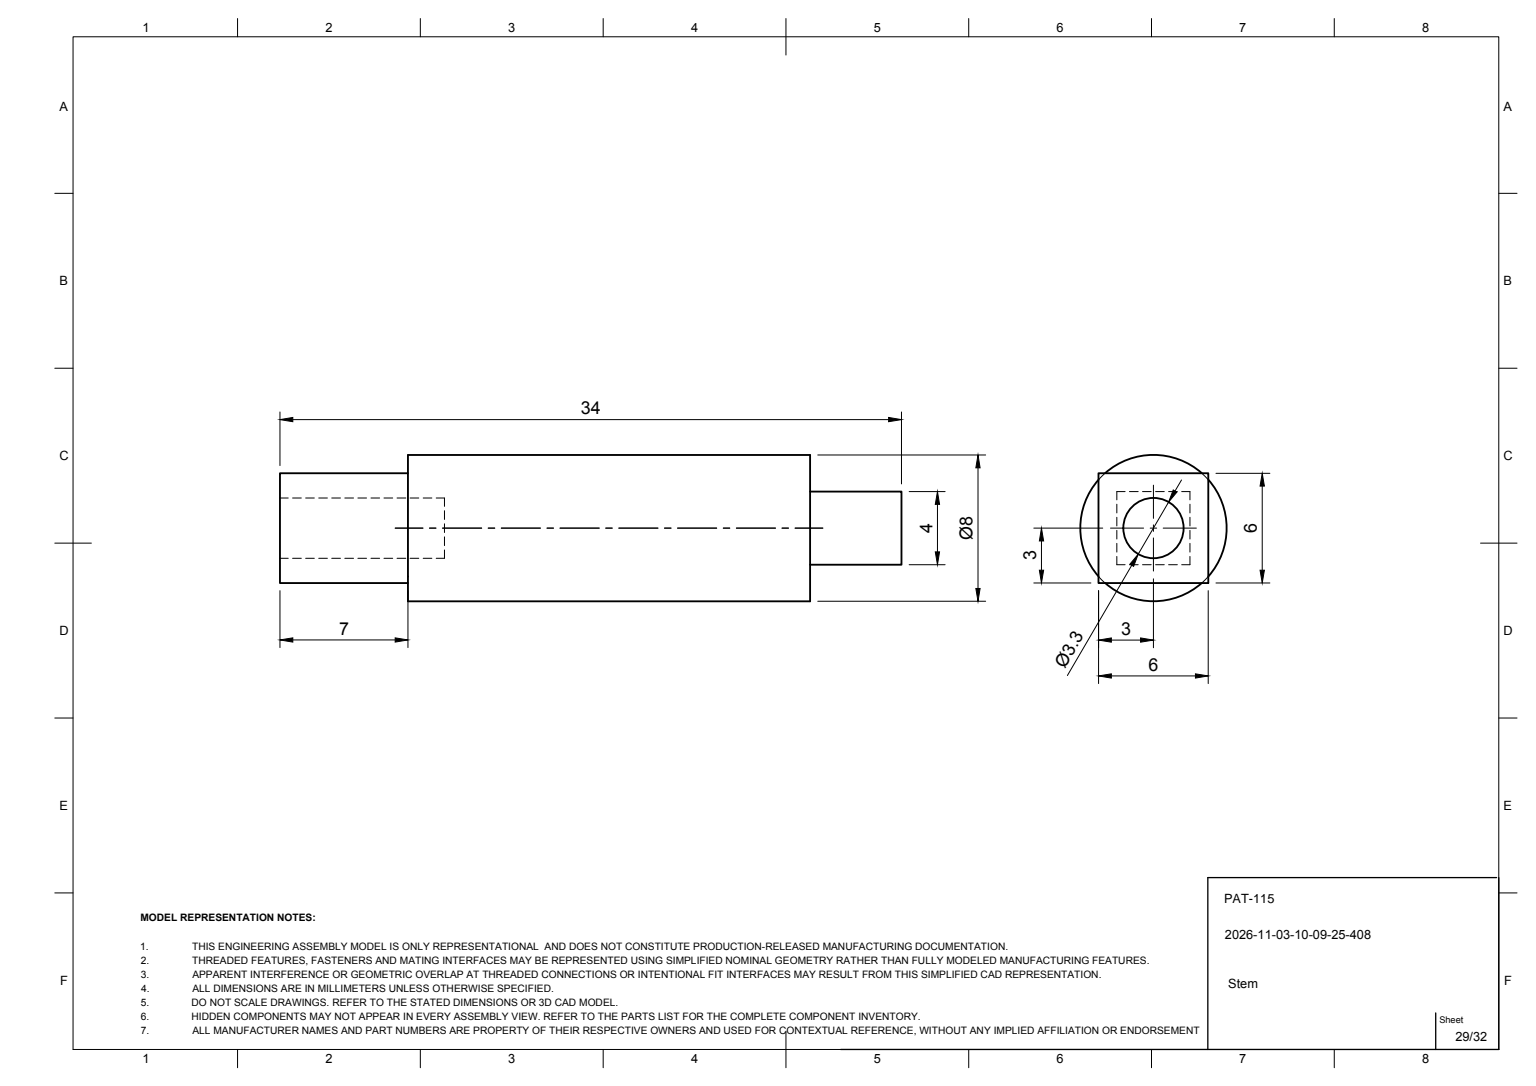
ISO-10303-21;
HEADER;
/* Generated by software containing ST-Developer
 * from STEP Tools, Inc. (www.steptools.com) 
 */

FILE_DESCRIPTION(
/* description */ ('Union bypass pipe loop'),
/* implementation_level */ '2;1');

FILE_NAME(
/* name */ 'Stem.step',
/* time_stamp */ '2026-10-27T21:00:29-07:00',
/* author */ (''),
/* organization */ (''),
/* preprocessor_version */ 'ST-DEVELOPER v20.2',
/* originating_system */ 'Autodesk Translation Framework v15.17.0.0',
/* authorisation */ '');

FILE_SCHEMA (('AUTOMOTIVE_DESIGN { 1 0 10303 214 3 1 1 }'));
ENDSEC;

DATA;
#10=MECHANICAL_DESIGN_GEOMETRIC_PRESENTATION_REPRESENTATION('',(#472),#10095);
#408=SHAPE_REPRESENTATION_RELATIONSHIP('SRR','None',#10278,#440);
#440=ADVANCED_BREP_SHAPE_REPRESENTATION('',(#501),#10090);
#472=STYLED_ITEM('',(#10493),#501);
#501=MANIFOLD_SOLID_BREP('Body1',#5546);
#628=FACE_BOUND('',#1569,.T.);
#629=FACE_BOUND('',#1581,.T.);
#786=PLANE('',#6529);
#787=PLANE('',#6530);
#788=PLANE('',#6532);
#789=PLANE('',#6534);
#790=PLANE('',#6536);
#791=PLANE('',#6538);
#792=PLANE('',#6539);
#793=PLANE('',#6540);
#794=PLANE('',#6541);
#795=PLANE('',#6542);
#796=PLANE('',#6543);
#797=PLANE('',#6545);
#798=PLANE('',#6548);
#799=PLANE('',#6550);
#800=PLANE('',#6552);
#801=PLANE('',#6553);
#802=PLANE('',#6554);
#803=PLANE('',#6555);
#804=PLANE('',#6556);
#805=PLANE('',#6559);
#1109=FACE_OUTER_BOUND('',#1558,.T.);
#1110=FACE_OUTER_BOUND('',#1559,.T.);
#1111=FACE_OUTER_BOUND('',#1560,.T.);
#1112=FACE_OUTER_BOUND('',#1561,.T.);
#1113=FACE_OUTER_BOUND('',#1562,.T.);
#1114=FACE_OUTER_BOUND('',#1563,.T.);
#1115=FACE_OUTER_BOUND('',#1564,.T.);
#1116=FACE_OUTER_BOUND('',#1565,.T.);
#1117=FACE_OUTER_BOUND('',#1566,.T.);
#1118=FACE_OUTER_BOUND('',#1567,.T.);
#1119=FACE_OUTER_BOUND('',#1568,.T.);
#1120=FACE_OUTER_BOUND('',#1570,.T.);
#1121=FACE_OUTER_BOUND('',#1571,.T.);
#1122=FACE_OUTER_BOUND('',#1572,.T.);
#1123=FACE_OUTER_BOUND('',#1573,.T.);
#1124=FACE_OUTER_BOUND('',#1574,.T.);
#1125=FACE_OUTER_BOUND('',#1575,.T.);
#1126=FACE_OUTER_BOUND('',#1576,.T.);
#1127=FACE_OUTER_BOUND('',#1577,.T.);
#1128=FACE_OUTER_BOUND('',#1578,.T.);
#1129=FACE_OUTER_BOUND('',#1579,.T.);
#1130=FACE_OUTER_BOUND('',#1580,.T.);
#1558=EDGE_LOOP('',(#4844,#4845,#4846,#4847));
#1559=EDGE_LOOP('',(#4848));
#1560=EDGE_LOOP('',(#4849,#4850,#4851));
#1561=EDGE_LOOP('',(#4852,#4853,#4854));
#1562=EDGE_LOOP('',(#4855,#4856,#4857));
#1563=EDGE_LOOP('',(#4858,#4859,#4860));
#1564=EDGE_LOOP('',(#4861,#4862,#4863,#4864,#4865,#4866));
#1565=EDGE_LOOP('',(#4867,#4868,#4869,#4870,#4871,#4872));
#1566=EDGE_LOOP('',(#4873,#4874,#4875,#4876,#4877,#4878));
#1567=EDGE_LOOP('',(#4879,#4880,#4881,#4882,#4883,#4884));
#1568=EDGE_LOOP('',(#4885,#4886,#4887,#4888));
#1569=EDGE_LOOP('',(#4889));
#1570=EDGE_LOOP('',(#4890,#4891));
#1571=EDGE_LOOP('',(#4892,#4893,#4894));
#1572=EDGE_LOOP('',(#4895,#4896));
#1573=EDGE_LOOP('',(#4897,#4898));
#1574=EDGE_LOOP('',(#4899,#4900,#4901,#4902));
#1575=EDGE_LOOP('',(#4903,#4904,#4905,#4906));
#1576=EDGE_LOOP('',(#4907,#4908,#4909,#4910));
#1577=EDGE_LOOP('',(#4911,#4912,#4913,#4914));
#1578=EDGE_LOOP('',(#4915,#4916,#4917,#4918));
#1579=EDGE_LOOP('',(#4919,#4920,#4921,#4922,#4923,#4924,#4925,#4926,#4927,
#4928,#4929,#4930));
#1580=EDGE_LOOP('',(#4931));
#1581=EDGE_LOOP('',(#4932,#4933,#4934,#4935));
#1904=LINE('',#9763,#2280);
#1905=LINE('',#9771,#2281);
#1906=LINE('',#9772,#2282);
#1907=LINE('',#9778,#2283);
#1908=LINE('',#9779,#2284);
#1909=LINE('',#9785,#2285);
#1910=LINE('',#9786,#2286);
#1911=LINE('',#9792,#2287);
#1912=LINE('',#9793,#2288);
#1913=LINE('',#9795,#2289);
#1914=LINE('',#9797,#2290);
#1915=LINE('',#9799,#2291);
#1916=LINE('',#9800,#2292);
#1917=LINE('',#9802,#2293);
#1918=LINE('',#9804,#2294);
#1919=LINE('',#9805,#2295);
#1920=LINE('',#9807,#2296);
#1921=LINE('',#9809,#2297);
#1922=LINE('',#9810,#2298);
#1923=LINE('',#9812,#2299);
#1924=LINE('',#9813,#2300);
#1925=LINE('',#9828,#2301);
#1926=LINE('',#9830,#2302);
#1927=LINE('',#9832,#2303);
#1928=LINE('',#9833,#2304);
#1929=LINE('',#9836,#2305);
#1930=LINE('',#9838,#2306);
#1931=LINE('',#9839,#2307);
#1932=LINE('',#9842,#2308);
#1933=LINE('',#9844,#2309);
#1934=LINE('',#9845,#2310);
#1935=LINE('',#9847,#2311);
#1936=LINE('',#9848,#2312);
#1937=LINE('',#9852,#2313);
#2280=VECTOR('',#8146,0.165);
#2281=VECTOR('',#8155,1.);
#2282=VECTOR('',#8156,1.);
#2283=VECTOR('',#8161,1.);
#2284=VECTOR('',#8162,1.);
#2285=VECTOR('',#8167,1.);
#2286=VECTOR('',#8168,1.);
#2287=VECTOR('',#8173,1.);
#2288=VECTOR('',#8174,1.);
#2289=VECTOR('',#8177,1.);
#2290=VECTOR('',#8178,1.);
#2291=VECTOR('',#8179,1.);
#2292=VECTOR('',#8180,1.);
#2293=VECTOR('',#8183,1.);
#2294=VECTOR('',#8184,1.);
#2295=VECTOR('',#8185,1.);
#2296=VECTOR('',#8188,1.);
#2297=VECTOR('',#8189,1.);
#2298=VECTOR('',#8190,1.);
#2299=VECTOR('',#8193,1.);
#2300=VECTOR('',#8194,1.);
#2301=VECTOR('',#8217,1.);
#2302=VECTOR('',#8218,1.);
#2303=VECTOR('',#8219,1.);
#2304=VECTOR('',#8220,1.);
#2305=VECTOR('',#8223,1.);
#2306=VECTOR('',#8224,1.);
#2307=VECTOR('',#8225,1.);
#2308=VECTOR('',#8228,1.);
#2309=VECTOR('',#8229,1.);
#2310=VECTOR('',#8230,1.);
#2311=VECTOR('',#8233,1.);
#2312=VECTOR('',#8234,1.);
#2313=VECTOR('',#8239,0.4);
#2607=CIRCLE('',#6527,0.165);
#2608=CIRCLE('',#6528,0.165);
#2609=CIRCLE('',#6531,0.4);
#2610=CIRCLE('',#6533,0.4);
#2611=CIRCLE('',#6535,0.4);
#2612=CIRCLE('',#6537,0.4);
#2613=CIRCLE('',#6544,0.4);
#2614=CIRCLE('',#6546,0.4);
#2615=CIRCLE('',#6547,0.4);
#2616=CIRCLE('',#6549,0.4);
#2617=CIRCLE('',#6551,0.4);
#2618=CIRCLE('',#6558,0.4);
#2992=VERTEX_POINT('',#9760);
#2993=VERTEX_POINT('',#9762);
#2994=VERTEX_POINT('',#9767);
#2995=VERTEX_POINT('',#9768);
#2996=VERTEX_POINT('',#9770);
#2997=VERTEX_POINT('',#9774);
#2998=VERTEX_POINT('',#9775);
#2999=VERTEX_POINT('',#9777);
#3000=VERTEX_POINT('',#9781);
#3001=VERTEX_POINT('',#9782);
#3002=VERTEX_POINT('',#9784);
#3003=VERTEX_POINT('',#9788);
#3004=VERTEX_POINT('',#9789);
#3005=VERTEX_POINT('',#9791);
#3006=VERTEX_POINT('',#9796);
#3007=VERTEX_POINT('',#9798);
#3008=VERTEX_POINT('',#9803);
#3009=VERTEX_POINT('',#9808);
#3010=VERTEX_POINT('',#9818);
#3011=VERTEX_POINT('',#9826);
#3012=VERTEX_POINT('',#9827);
#3013=VERTEX_POINT('',#9829);
#3014=VERTEX_POINT('',#9831);
#3015=VERTEX_POINT('',#9835);
#3016=VERTEX_POINT('',#9837);
#3017=VERTEX_POINT('',#9841);
#3018=VERTEX_POINT('',#9843);
#3019=VERTEX_POINT('',#9851);
#3620=EDGE_CURVE('',#2992,#2992,#2607,.T.);
#3621=EDGE_CURVE('',#2992,#2993,#1904,.T.);
#3622=EDGE_CURVE('',#2993,#2993,#2608,.T.);
#3623=EDGE_CURVE('',#2994,#2995,#2609,.T.);
#3624=EDGE_CURVE('',#2996,#2995,#1905,.T.);
#3625=EDGE_CURVE('',#2994,#2996,#1906,.T.);
#3626=EDGE_CURVE('',#2997,#2998,#2610,.T.);
#3627=EDGE_CURVE('',#2999,#2998,#1907,.T.);
#3628=EDGE_CURVE('',#2997,#2999,#1908,.T.);
#3629=EDGE_CURVE('',#3000,#3001,#2611,.T.);
#3630=EDGE_CURVE('',#3002,#3001,#1909,.T.);
#3631=EDGE_CURVE('',#3000,#3002,#1910,.T.);
#3632=EDGE_CURVE('',#3003,#3004,#2612,.T.);
#3633=EDGE_CURVE('',#3005,#3004,#1911,.T.);
#3634=EDGE_CURVE('',#3003,#3005,#1912,.T.);
#3635=EDGE_CURVE('',#2994,#3004,#1913,.T.);
#3636=EDGE_CURVE('',#2996,#3006,#1914,.T.);
#3637=EDGE_CURVE('',#3007,#3006,#1915,.T.);
#3638=EDGE_CURVE('',#3005,#3007,#1916,.T.);
#3639=EDGE_CURVE('',#3003,#3001,#1917,.T.);
#3640=EDGE_CURVE('',#3008,#3007,#1918,.T.);
#3641=EDGE_CURVE('',#3002,#3008,#1919,.T.);
#3642=EDGE_CURVE('',#3000,#2998,#1920,.T.);
#3643=EDGE_CURVE('',#3009,#3008,#1921,.T.);
#3644=EDGE_CURVE('',#2999,#3009,#1922,.T.);
#3645=EDGE_CURVE('',#2997,#2995,#1923,.T.);
#3646=EDGE_CURVE('',#3006,#3009,#1924,.T.);
#3647=EDGE_CURVE('',#2998,#3000,#2613,.T.);
#3648=EDGE_CURVE('',#2995,#3010,#2614,.T.);
#3649=EDGE_CURVE('',#3010,#2997,#2615,.T.);
#3650=EDGE_CURVE('',#3004,#2994,#2616,.T.);
#3651=EDGE_CURVE('',#3001,#3003,#2617,.T.);
#3652=EDGE_CURVE('',#3011,#3012,#1925,.T.);
#3653=EDGE_CURVE('',#3012,#3013,#1926,.T.);
#3654=EDGE_CURVE('',#3014,#3013,#1927,.T.);
#3655=EDGE_CURVE('',#3011,#3014,#1928,.T.);
#3656=EDGE_CURVE('',#3015,#3011,#1929,.T.);
#3657=EDGE_CURVE('',#3016,#3014,#1930,.T.);
#3658=EDGE_CURVE('',#3015,#3016,#1931,.T.);
#3659=EDGE_CURVE('',#3017,#3015,#1932,.T.);
#3660=EDGE_CURVE('',#3018,#3016,#1933,.T.);
#3661=EDGE_CURVE('',#3017,#3018,#1934,.T.);
#3662=EDGE_CURVE('',#3012,#3017,#1935,.T.);
#3663=EDGE_CURVE('',#3013,#3018,#1936,.T.);
#3664=EDGE_CURVE('',#3010,#3019,#1937,.T.);
#3665=EDGE_CURVE('',#3019,#3019,#2618,.T.);
#4844=ORIENTED_EDGE('',*,*,#3620,.F.);
#4845=ORIENTED_EDGE('',*,*,#3621,.T.);
#4846=ORIENTED_EDGE('',*,*,#3622,.F.);
#4847=ORIENTED_EDGE('',*,*,#3621,.F.);
#4848=ORIENTED_EDGE('',*,*,#3620,.T.);
#4849=ORIENTED_EDGE('',*,*,#3623,.T.);
#4850=ORIENTED_EDGE('',*,*,#3624,.F.);
#4851=ORIENTED_EDGE('',*,*,#3625,.F.);
#4852=ORIENTED_EDGE('',*,*,#3626,.T.);
#4853=ORIENTED_EDGE('',*,*,#3627,.F.);
#4854=ORIENTED_EDGE('',*,*,#3628,.F.);
#4855=ORIENTED_EDGE('',*,*,#3629,.T.);
#4856=ORIENTED_EDGE('',*,*,#3630,.F.);
#4857=ORIENTED_EDGE('',*,*,#3631,.F.);
#4858=ORIENTED_EDGE('',*,*,#3632,.T.);
#4859=ORIENTED_EDGE('',*,*,#3633,.F.);
#4860=ORIENTED_EDGE('',*,*,#3634,.F.);
#4861=ORIENTED_EDGE('',*,*,#3633,.T.);
#4862=ORIENTED_EDGE('',*,*,#3635,.F.);
#4863=ORIENTED_EDGE('',*,*,#3625,.T.);
#4864=ORIENTED_EDGE('',*,*,#3636,.T.);
#4865=ORIENTED_EDGE('',*,*,#3637,.F.);
#4866=ORIENTED_EDGE('',*,*,#3638,.F.);
#4867=ORIENTED_EDGE('',*,*,#3630,.T.);
#4868=ORIENTED_EDGE('',*,*,#3639,.F.);
#4869=ORIENTED_EDGE('',*,*,#3634,.T.);
#4870=ORIENTED_EDGE('',*,*,#3638,.T.);
#4871=ORIENTED_EDGE('',*,*,#3640,.F.);
#4872=ORIENTED_EDGE('',*,*,#3641,.F.);
#4873=ORIENTED_EDGE('',*,*,#3627,.T.);
#4874=ORIENTED_EDGE('',*,*,#3642,.F.);
#4875=ORIENTED_EDGE('',*,*,#3631,.T.);
#4876=ORIENTED_EDGE('',*,*,#3641,.T.);
#4877=ORIENTED_EDGE('',*,*,#3643,.F.);
#4878=ORIENTED_EDGE('',*,*,#3644,.F.);
#4879=ORIENTED_EDGE('',*,*,#3624,.T.);
#4880=ORIENTED_EDGE('',*,*,#3645,.F.);
#4881=ORIENTED_EDGE('',*,*,#3628,.T.);
#4882=ORIENTED_EDGE('',*,*,#3644,.T.);
#4883=ORIENTED_EDGE('',*,*,#3646,.F.);
#4884=ORIENTED_EDGE('',*,*,#3636,.F.);
#4885=ORIENTED_EDGE('',*,*,#3646,.T.);
#4886=ORIENTED_EDGE('',*,*,#3643,.T.);
#4887=ORIENTED_EDGE('',*,*,#3640,.T.);
#4888=ORIENTED_EDGE('',*,*,#3637,.T.);
#4889=ORIENTED_EDGE('',*,*,#3622,.T.);
#4890=ORIENTED_EDGE('',*,*,#3642,.T.);
#4891=ORIENTED_EDGE('',*,*,#3647,.T.);
#4892=ORIENTED_EDGE('',*,*,#3645,.T.);
#4893=ORIENTED_EDGE('',*,*,#3648,.T.);
#4894=ORIENTED_EDGE('',*,*,#3649,.T.);
#4895=ORIENTED_EDGE('',*,*,#3635,.T.);
#4896=ORIENTED_EDGE('',*,*,#3650,.T.);
#4897=ORIENTED_EDGE('',*,*,#3639,.T.);
#4898=ORIENTED_EDGE('',*,*,#3651,.T.);
#4899=ORIENTED_EDGE('',*,*,#3652,.T.);
#4900=ORIENTED_EDGE('',*,*,#3653,.T.);
#4901=ORIENTED_EDGE('',*,*,#3654,.F.);
#4902=ORIENTED_EDGE('',*,*,#3655,.F.);
#4903=ORIENTED_EDGE('',*,*,#3656,.T.);
#4904=ORIENTED_EDGE('',*,*,#3655,.T.);
#4905=ORIENTED_EDGE('',*,*,#3657,.F.);
#4906=ORIENTED_EDGE('',*,*,#3658,.F.);
#4907=ORIENTED_EDGE('',*,*,#3659,.T.);
#4908=ORIENTED_EDGE('',*,*,#3658,.T.);
#4909=ORIENTED_EDGE('',*,*,#3660,.F.);
#4910=ORIENTED_EDGE('',*,*,#3661,.F.);
#4911=ORIENTED_EDGE('',*,*,#3662,.T.);
#4912=ORIENTED_EDGE('',*,*,#3661,.T.);
#4913=ORIENTED_EDGE('',*,*,#3663,.F.);
#4914=ORIENTED_EDGE('',*,*,#3653,.F.);
#4915=ORIENTED_EDGE('',*,*,#3662,.F.);
#4916=ORIENTED_EDGE('',*,*,#3652,.F.);
#4917=ORIENTED_EDGE('',*,*,#3656,.F.);
#4918=ORIENTED_EDGE('',*,*,#3659,.F.);
#4919=ORIENTED_EDGE('',*,*,#3648,.F.);
#4920=ORIENTED_EDGE('',*,*,#3623,.F.);
#4921=ORIENTED_EDGE('',*,*,#3650,.F.);
#4922=ORIENTED_EDGE('',*,*,#3632,.F.);
#4923=ORIENTED_EDGE('',*,*,#3651,.F.);
#4924=ORIENTED_EDGE('',*,*,#3629,.F.);
#4925=ORIENTED_EDGE('',*,*,#3647,.F.);
#4926=ORIENTED_EDGE('',*,*,#3626,.F.);
#4927=ORIENTED_EDGE('',*,*,#3649,.F.);
#4928=ORIENTED_EDGE('',*,*,#3664,.T.);
#4929=ORIENTED_EDGE('',*,*,#3665,.T.);
#4930=ORIENTED_EDGE('',*,*,#3664,.F.);
#4931=ORIENTED_EDGE('',*,*,#3665,.F.);
#4932=ORIENTED_EDGE('',*,*,#3654,.T.);
#4933=ORIENTED_EDGE('',*,*,#3663,.T.);
#4934=ORIENTED_EDGE('',*,*,#3660,.T.);
#4935=ORIENTED_EDGE('',*,*,#3657,.T.);
#5178=CYLINDRICAL_SURFACE('',#6526,0.165);
#5179=CYLINDRICAL_SURFACE('',#6557,0.4);
#5458=ADVANCED_FACE('',(#1109),#5178,.F.);
#5459=ADVANCED_FACE('',(#1110),#786,.T.);
#5460=ADVANCED_FACE('',(#1111),#787,.F.);
#5461=ADVANCED_FACE('',(#1112),#788,.F.);
#5462=ADVANCED_FACE('',(#1113),#789,.F.);
#5463=ADVANCED_FACE('',(#1114),#790,.F.);
#5464=ADVANCED_FACE('',(#1115),#791,.T.);
#5465=ADVANCED_FACE('',(#1116),#792,.T.);
#5466=ADVANCED_FACE('',(#1117),#793,.T.);
#5467=ADVANCED_FACE('',(#1118),#794,.T.);
#5468=ADVANCED_FACE('',(#1119,#628),#795,.T.);
#5469=ADVANCED_FACE('',(#1120),#796,.T.);
#5470=ADVANCED_FACE('',(#1121),#797,.T.);
#5471=ADVANCED_FACE('',(#1122),#798,.T.);
#5472=ADVANCED_FACE('',(#1123),#799,.T.);
#5473=ADVANCED_FACE('',(#1124),#800,.T.);
#5474=ADVANCED_FACE('',(#1125),#801,.T.);
#5475=ADVANCED_FACE('',(#1126),#802,.T.);
#5476=ADVANCED_FACE('',(#1127),#803,.T.);
#5477=ADVANCED_FACE('',(#1128),#804,.F.);
#5478=ADVANCED_FACE('',(#1129),#5179,.T.);
#5479=ADVANCED_FACE('',(#1130,#629),#805,.F.);
#5546=CLOSED_SHELL('',(#5458,#5459,#5460,#5461,#5462,#5463,#5464,#5465,
#5466,#5467,#5468,#5469,#5470,#5471,#5472,#5473,#5474,#5475,#5476,#5477,
#5478,#5479));
#6525=AXIS2_PLACEMENT_3D('',#9758,#8140,#8141);
#6526=AXIS2_PLACEMENT_3D('',#9759,#8142,#8143);
#6527=AXIS2_PLACEMENT_3D('',#9761,#8144,#8145);
#6528=AXIS2_PLACEMENT_3D('',#9764,#8147,#8148);
#6529=AXIS2_PLACEMENT_3D('',#9765,#8149,#8150);
#6530=AXIS2_PLACEMENT_3D('',#9766,#8151,#8152);
#6531=AXIS2_PLACEMENT_3D('',#9769,#8153,#8154);
#6532=AXIS2_PLACEMENT_3D('',#9773,#8157,#8158);
#6533=AXIS2_PLACEMENT_3D('',#9776,#8159,#8160);
#6534=AXIS2_PLACEMENT_3D('',#9780,#8163,#8164);
#6535=AXIS2_PLACEMENT_3D('',#9783,#8165,#8166);
#6536=AXIS2_PLACEMENT_3D('',#9787,#8169,#8170);
#6537=AXIS2_PLACEMENT_3D('',#9790,#8171,#8172);
#6538=AXIS2_PLACEMENT_3D('',#9794,#8175,#8176);
#6539=AXIS2_PLACEMENT_3D('',#9801,#8181,#8182);
#6540=AXIS2_PLACEMENT_3D('',#9806,#8186,#8187);
#6541=AXIS2_PLACEMENT_3D('',#9811,#8191,#8192);
#6542=AXIS2_PLACEMENT_3D('',#9814,#8195,#8196);
#6543=AXIS2_PLACEMENT_3D('',#9815,#8197,#8198);
#6544=AXIS2_PLACEMENT_3D('',#9816,#8199,#8200);
#6545=AXIS2_PLACEMENT_3D('',#9817,#8201,#8202);
#6546=AXIS2_PLACEMENT_3D('',#9819,#8203,#8204);
#6547=AXIS2_PLACEMENT_3D('',#9820,#8205,#8206);
#6548=AXIS2_PLACEMENT_3D('',#9821,#8207,#8208);
#6549=AXIS2_PLACEMENT_3D('',#9822,#8209,#8210);
#6550=AXIS2_PLACEMENT_3D('',#9823,#8211,#8212);
#6551=AXIS2_PLACEMENT_3D('',#9824,#8213,#8214);
#6552=AXIS2_PLACEMENT_3D('',#9825,#8215,#8216);
#6553=AXIS2_PLACEMENT_3D('',#9834,#8221,#8222);
#6554=AXIS2_PLACEMENT_3D('',#9840,#8226,#8227);
#6555=AXIS2_PLACEMENT_3D('',#9846,#8231,#8232);
#6556=AXIS2_PLACEMENT_3D('',#9849,#8235,#8236);
#6557=AXIS2_PLACEMENT_3D('',#9850,#8237,#8238);
#6558=AXIS2_PLACEMENT_3D('',#9853,#8240,#8241);
#6559=AXIS2_PLACEMENT_3D('',#9854,#8242,#8243);
#8140=DIRECTION('axis',(0.,0.,1.));
#8141=DIRECTION('refdir',(1.,0.,0.));
#8142=DIRECTION('center_axis',(0.,0.,1.));
#8143=DIRECTION('ref_axis',(1.,0.,0.));
#8144=DIRECTION('center_axis',(0.,0.,1.));
#8145=DIRECTION('ref_axis',(1.,0.,0.));
#8146=DIRECTION('',(0.,0.,1.));
#8147=DIRECTION('center_axis',(0.,0.,-1.));
#8148=DIRECTION('ref_axis',(1.,0.,0.));
#8149=DIRECTION('center_axis',(0.,0.,1.));
#8150=DIRECTION('ref_axis',(1.,0.,0.));
#8151=DIRECTION('center_axis',(0.,0.,1.));
#8152=DIRECTION('ref_axis',(1.,0.,0.));
#8153=DIRECTION('center_axis',(0.,0.,1.));
#8154=DIRECTION('ref_axis',(1.,0.,0.));
#8155=DIRECTION('',(0.,-1.,0.));
#8156=DIRECTION('',(-1.,0.,0.));
#8157=DIRECTION('center_axis',(0.,0.,1.));
#8158=DIRECTION('ref_axis',(1.,0.,0.));
#8159=DIRECTION('center_axis',(0.,0.,1.));
#8160=DIRECTION('ref_axis',(1.,0.,0.));
#8161=DIRECTION('',(1.,0.,0.));
#8162=DIRECTION('',(0.,-1.,0.));
#8163=DIRECTION('center_axis',(0.,0.,1.));
#8164=DIRECTION('ref_axis',(1.,0.,0.));
#8165=DIRECTION('center_axis',(0.,0.,1.));
#8166=DIRECTION('ref_axis',(1.,0.,0.));
#8167=DIRECTION('',(0.,1.,0.));
#8168=DIRECTION('',(1.,0.,0.));
#8169=DIRECTION('center_axis',(0.,0.,1.));
#8170=DIRECTION('ref_axis',(1.,0.,0.));
#8171=DIRECTION('center_axis',(0.,0.,1.));
#8172=DIRECTION('ref_axis',(1.,0.,0.));
#8173=DIRECTION('',(-1.,0.,0.));
#8174=DIRECTION('',(0.,1.,0.));
#8175=DIRECTION('center_axis',(0.,1.,0.));
#8176=DIRECTION('ref_axis',(-1.,0.,0.));
#8177=DIRECTION('',(1.,0.,0.));
#8178=DIRECTION('',(0.,0.,1.));
#8179=DIRECTION('',(-1.,0.,0.));
#8180=DIRECTION('',(0.,0.,1.));
#8181=DIRECTION('center_axis',(1.,0.,0.));
#8182=DIRECTION('ref_axis',(0.,1.,0.));
#8183=DIRECTION('',(0.,-1.,0.));
#8184=DIRECTION('',(0.,1.,0.));
#8185=DIRECTION('',(0.,0.,1.));
#8186=DIRECTION('center_axis',(0.,-1.,0.));
#8187=DIRECTION('ref_axis',(1.,0.,0.));
#8188=DIRECTION('',(-1.,0.,0.));
#8189=DIRECTION('',(1.,0.,0.));
#8190=DIRECTION('',(0.,0.,1.));
#8191=DIRECTION('center_axis',(-1.,0.,0.));
#8192=DIRECTION('ref_axis',(0.,-1.,0.));
#8193=DIRECTION('',(0.,1.,0.));
#8194=DIRECTION('',(0.,-1.,0.));
#8195=DIRECTION('center_axis',(0.,0.,1.));
#8196=DIRECTION('ref_axis',(1.,0.,0.));
#8197=DIRECTION('center_axis',(0.,0.,1.));
#8198=DIRECTION('ref_axis',(1.,0.,0.));
#8199=DIRECTION('center_axis',(0.,0.,1.));
#8200=DIRECTION('ref_axis',(1.,0.,0.));
#8201=DIRECTION('center_axis',(0.,0.,1.));
#8202=DIRECTION('ref_axis',(1.,0.,0.));
#8203=DIRECTION('center_axis',(0.,0.,1.));
#8204=DIRECTION('ref_axis',(1.,0.,0.));
#8205=DIRECTION('center_axis',(0.,0.,1.));
#8206=DIRECTION('ref_axis',(1.,0.,0.));
#8207=DIRECTION('center_axis',(0.,0.,1.));
#8208=DIRECTION('ref_axis',(1.,0.,0.));
#8209=DIRECTION('center_axis',(0.,0.,1.));
#8210=DIRECTION('ref_axis',(1.,0.,0.));
#8211=DIRECTION('center_axis',(0.,0.,1.));
#8212=DIRECTION('ref_axis',(1.,0.,0.));
#8213=DIRECTION('center_axis',(0.,0.,1.));
#8214=DIRECTION('ref_axis',(1.,0.,0.));
#8215=DIRECTION('center_axis',(0.,1.,0.));
#8216=DIRECTION('ref_axis',(-1.,0.,0.));
#8217=DIRECTION('',(-1.,0.,0.));
#8218=DIRECTION('',(0.,0.,1.));
#8219=DIRECTION('',(-1.,0.,0.));
#8220=DIRECTION('',(0.,0.,1.));
#8221=DIRECTION('center_axis',(1.,0.,0.));
#8222=DIRECTION('ref_axis',(0.,1.,0.));
#8223=DIRECTION('',(0.,1.,0.));
#8224=DIRECTION('',(0.,1.,0.));
#8225=DIRECTION('',(0.,0.,1.));
#8226=DIRECTION('center_axis',(0.,-1.,0.));
#8227=DIRECTION('ref_axis',(1.,0.,0.));
#8228=DIRECTION('',(1.,0.,0.));
#8229=DIRECTION('',(1.,0.,0.));
#8230=DIRECTION('',(0.,0.,1.));
#8231=DIRECTION('center_axis',(-1.,0.,0.));
#8232=DIRECTION('ref_axis',(0.,-1.,0.));
#8233=DIRECTION('',(0.,-1.,0.));
#8234=DIRECTION('',(0.,-1.,0.));
#8235=DIRECTION('center_axis',(0.,0.,1.));
#8236=DIRECTION('ref_axis',(1.,0.,0.));
#8237=DIRECTION('center_axis',(0.,0.,1.));
#8238=DIRECTION('ref_axis',(1.,0.,0.));
#8239=DIRECTION('',(0.,0.,-1.));
#8240=DIRECTION('center_axis',(0.,0.,1.));
#8241=DIRECTION('ref_axis',(1.,0.,0.));
#8242=DIRECTION('center_axis',(0.,0.,1.));
#8243=DIRECTION('ref_axis',(1.,0.,0.));
#9758=CARTESIAN_POINT('',(0.,0.,0.));
#9759=CARTESIAN_POINT('Origin',(0.,0.,8.5));
#9760=CARTESIAN_POINT('',(-0.165,-2.02066721859313E-17,8.5));
#9761=CARTESIAN_POINT('Origin',(0.,0.,8.5));
#9762=CARTESIAN_POINT('',(-0.165,2.02066721859313E-17,9.4));
#9763=CARTESIAN_POINT('',(-0.165,-2.02066721859313E-17,8.5));
#9764=CARTESIAN_POINT('Origin',(0.,0.,9.4));
#9765=CARTESIAN_POINT('Origin',(0.,0.,8.5));
#9766=CARTESIAN_POINT('Origin',(0.,0.,8.7));
#9767=CARTESIAN_POINT('',(-0.264575131106459,0.3,8.7));
#9768=CARTESIAN_POINT('',(-0.3,0.264575131106459,8.7));
#9769=CARTESIAN_POINT('Origin',(0.,0.,8.7));
#9770=CARTESIAN_POINT('',(-0.3,0.3,8.7));
#9771=CARTESIAN_POINT('',(-0.3,0.3,8.7));
#9772=CARTESIAN_POINT('',(0.3,0.3,8.7));
#9773=CARTESIAN_POINT('Origin',(0.,0.,8.7));
#9774=CARTESIAN_POINT('',(-0.3,-0.264575131106459,8.7));
#9775=CARTESIAN_POINT('',(-0.264575131106459,-0.3,8.7));
#9776=CARTESIAN_POINT('Origin',(0.,0.,8.7));
#9777=CARTESIAN_POINT('',(-0.3,-0.3,8.7));
#9778=CARTESIAN_POINT('',(-0.3,-0.3,8.7));
#9779=CARTESIAN_POINT('',(-0.3,0.3,8.7));
#9780=CARTESIAN_POINT('Origin',(0.,0.,8.7));
#9781=CARTESIAN_POINT('',(0.264575131106459,-0.3,8.7));
#9782=CARTESIAN_POINT('',(0.3,-0.264575131106459,8.7));
#9783=CARTESIAN_POINT('Origin',(0.,0.,8.7));
#9784=CARTESIAN_POINT('',(0.3,-0.3,8.7));
#9785=CARTESIAN_POINT('',(0.3,-0.3,8.7));
#9786=CARTESIAN_POINT('',(-0.3,-0.3,8.7));
#9787=CARTESIAN_POINT('Origin',(0.,0.,8.7));
#9788=CARTESIAN_POINT('',(0.3,0.264575131106459,8.7));
#9789=CARTESIAN_POINT('',(0.264575131106459,0.3,8.7));
#9790=CARTESIAN_POINT('Origin',(0.,0.,8.7));
#9791=CARTESIAN_POINT('',(0.3,0.3,8.7));
#9792=CARTESIAN_POINT('',(0.3,0.3,8.7));
#9793=CARTESIAN_POINT('',(0.3,-0.3,8.7));
#9794=CARTESIAN_POINT('Origin',(0.3,0.3,8.7));
#9795=CARTESIAN_POINT('',(0.15,0.3,8.7));
#9796=CARTESIAN_POINT('',(-0.3,0.3,9.4));
#9797=CARTESIAN_POINT('',(-0.3,0.3,8.7));
#9798=CARTESIAN_POINT('',(0.3,0.3,9.4));
#9799=CARTESIAN_POINT('',(0.3,0.3,9.4));
#9800=CARTESIAN_POINT('',(0.3,0.3,8.7));
#9801=CARTESIAN_POINT('Origin',(0.3,-0.3,8.7));
#9802=CARTESIAN_POINT('',(0.3,-0.15,8.7));
#9803=CARTESIAN_POINT('',(0.3,-0.3,9.4));
#9804=CARTESIAN_POINT('',(0.3,-0.3,9.4));
#9805=CARTESIAN_POINT('',(0.3,-0.3,8.7));
#9806=CARTESIAN_POINT('Origin',(-0.3,-0.3,8.7));
#9807=CARTESIAN_POINT('',(-0.15,-0.3,8.7));
#9808=CARTESIAN_POINT('',(-0.3,-0.3,9.4));
#9809=CARTESIAN_POINT('',(-0.3,-0.3,9.4));
#9810=CARTESIAN_POINT('',(-0.3,-0.3,8.7));
#9811=CARTESIAN_POINT('Origin',(-0.3,0.3,8.7));
#9812=CARTESIAN_POINT('',(-0.3,0.15,8.7));
#9813=CARTESIAN_POINT('',(-0.3,0.3,9.4));
#9814=CARTESIAN_POINT('Origin',(0.,0.,9.4));
#9815=CARTESIAN_POINT('Origin',(0.,0.,8.7));
#9816=CARTESIAN_POINT('Origin',(0.,0.,8.7));
#9817=CARTESIAN_POINT('Origin',(0.,0.,8.7));
#9818=CARTESIAN_POINT('',(-0.4,-4.89858719658941E-17,8.7));
#9819=CARTESIAN_POINT('Origin',(0.,0.,8.7));
#9820=CARTESIAN_POINT('Origin',(0.,0.,8.7));
#9821=CARTESIAN_POINT('Origin',(0.,0.,8.7));
#9822=CARTESIAN_POINT('Origin',(0.,0.,8.7));
#9823=CARTESIAN_POINT('Origin',(0.,0.,8.7));
#9824=CARTESIAN_POINT('Origin',(0.,0.,8.7));
#9825=CARTESIAN_POINT('Origin',(0.2,0.2,6.));
#9826=CARTESIAN_POINT('',(0.2,0.2,6.));
#9827=CARTESIAN_POINT('',(-0.2,0.2,6.));
#9828=CARTESIAN_POINT('',(0.2,0.2,6.));
#9829=CARTESIAN_POINT('',(-0.2,0.2,6.5));
#9830=CARTESIAN_POINT('',(-0.2,0.2,6.));
#9831=CARTESIAN_POINT('',(0.2,0.2,6.5));
#9832=CARTESIAN_POINT('',(0.1,0.2,6.5));
#9833=CARTESIAN_POINT('',(0.2,0.2,6.));
#9834=CARTESIAN_POINT('Origin',(0.2,-0.2,6.));
#9835=CARTESIAN_POINT('',(0.2,-0.2,6.));
#9836=CARTESIAN_POINT('',(0.2,-0.2,6.));
#9837=CARTESIAN_POINT('',(0.2,-0.2,6.5));
#9838=CARTESIAN_POINT('',(0.2,-0.1,6.5));
#9839=CARTESIAN_POINT('',(0.2,-0.2,6.));
#9840=CARTESIAN_POINT('Origin',(-0.2,-0.2,6.));
#9841=CARTESIAN_POINT('',(-0.2,-0.2,6.));
#9842=CARTESIAN_POINT('',(-0.2,-0.2,6.));
#9843=CARTESIAN_POINT('',(-0.2,-0.2,6.5));
#9844=CARTESIAN_POINT('',(-0.1,-0.2,6.5));
#9845=CARTESIAN_POINT('',(-0.2,-0.2,6.));
#9846=CARTESIAN_POINT('Origin',(-0.2,0.2,6.));
#9847=CARTESIAN_POINT('',(-0.2,0.2,6.));
#9848=CARTESIAN_POINT('',(-0.2,0.1,6.5));
#9849=CARTESIAN_POINT('Origin',(0.,0.,6.));
#9850=CARTESIAN_POINT('Origin',(0.,0.,6.5));
#9851=CARTESIAN_POINT('',(-0.4,-4.89858719658941E-17,6.5));
#9852=CARTESIAN_POINT('',(-0.4,-4.89858719658941E-17,6.5));
#9853=CARTESIAN_POINT('Origin',(0.,0.,6.5));
#9854=CARTESIAN_POINT('Origin',(0.,0.,6.5));
#10053=UNCERTAINTY_MEASURE_WITH_UNIT(LENGTH_MEASURE(0.001),#10096,
'DISTANCE_ACCURACY_VALUE',
'Maximum model space distance between geometric entities at asserted c
onnectivities');
#10058=UNCERTAINTY_MEASURE_WITH_UNIT(LENGTH_MEASURE(0.001),#10096,
'DISTANCE_ACCURACY_VALUE',
'Maximum model space distance between geometric entities at asserted c
onnectivities');
#10090=(
GEOMETRIC_REPRESENTATION_CONTEXT(3)
GLOBAL_UNCERTAINTY_ASSIGNED_CONTEXT((#10053))
GLOBAL_UNIT_ASSIGNED_CONTEXT((#10096,#10098,#10099))
REPRESENTATION_CONTEXT('','3D')
);
#10095=(
GEOMETRIC_REPRESENTATION_CONTEXT(3)
GLOBAL_UNCERTAINTY_ASSIGNED_CONTEXT((#10058))
GLOBAL_UNIT_ASSIGNED_CONTEXT((#10096,#10098,#10099))
REPRESENTATION_CONTEXT('','3D')
);
#10096=(
LENGTH_UNIT()
NAMED_UNIT(*)
SI_UNIT(.CENTI.,.METRE.)
);
#10098=(
NAMED_UNIT(*)
PLANE_ANGLE_UNIT()
SI_UNIT($,.RADIAN.)
);
#10099=(
NAMED_UNIT(*)
SI_UNIT($,.STERADIAN.)
SOLID_ANGLE_UNIT()
);
#10131=SHAPE_DEFINITION_REPRESENTATION(#10234,#10278);
#10234=PRODUCT_DEFINITION_SHAPE('',$,#10315);
#10278=SHAPE_REPRESENTATION('',(#6525),#10090);
#10283=PRODUCT_DEFINITION_CONTEXT('part definition',#10393,'design');
#10315=PRODUCT_DEFINITION('Stem','Stem',#10351,#10283);
#10351=PRODUCT_DEFINITION_FORMATION('',$,#10426);
#10393=APPLICATION_CONTEXT(
'Core Data for Automotive Mechanical Design Process');
#10394=PRODUCT_CONTEXT('part definition',#10393,'mechanical');
#10426=PRODUCT('Stem','Stem','Stem',(#10394));
#10487=COLOUR_RGB('Sky Blue',0.24,0.69,0.87);
#10488=FILL_AREA_STYLE_COLOUR('',#10487);
#10489=FILL_AREA_STYLE('',(#10488));
#10490=SURFACE_STYLE_FILL_AREA(#10489);
#10491=SURFACE_SIDE_STYLE('',(#10490));
#10492=SURFACE_STYLE_USAGE(.BOTH.,#10491);
#10493=PRESENTATION_STYLE_ASSIGNMENT((#10492));
ENDSEC;
END-ISO-10303-21;
